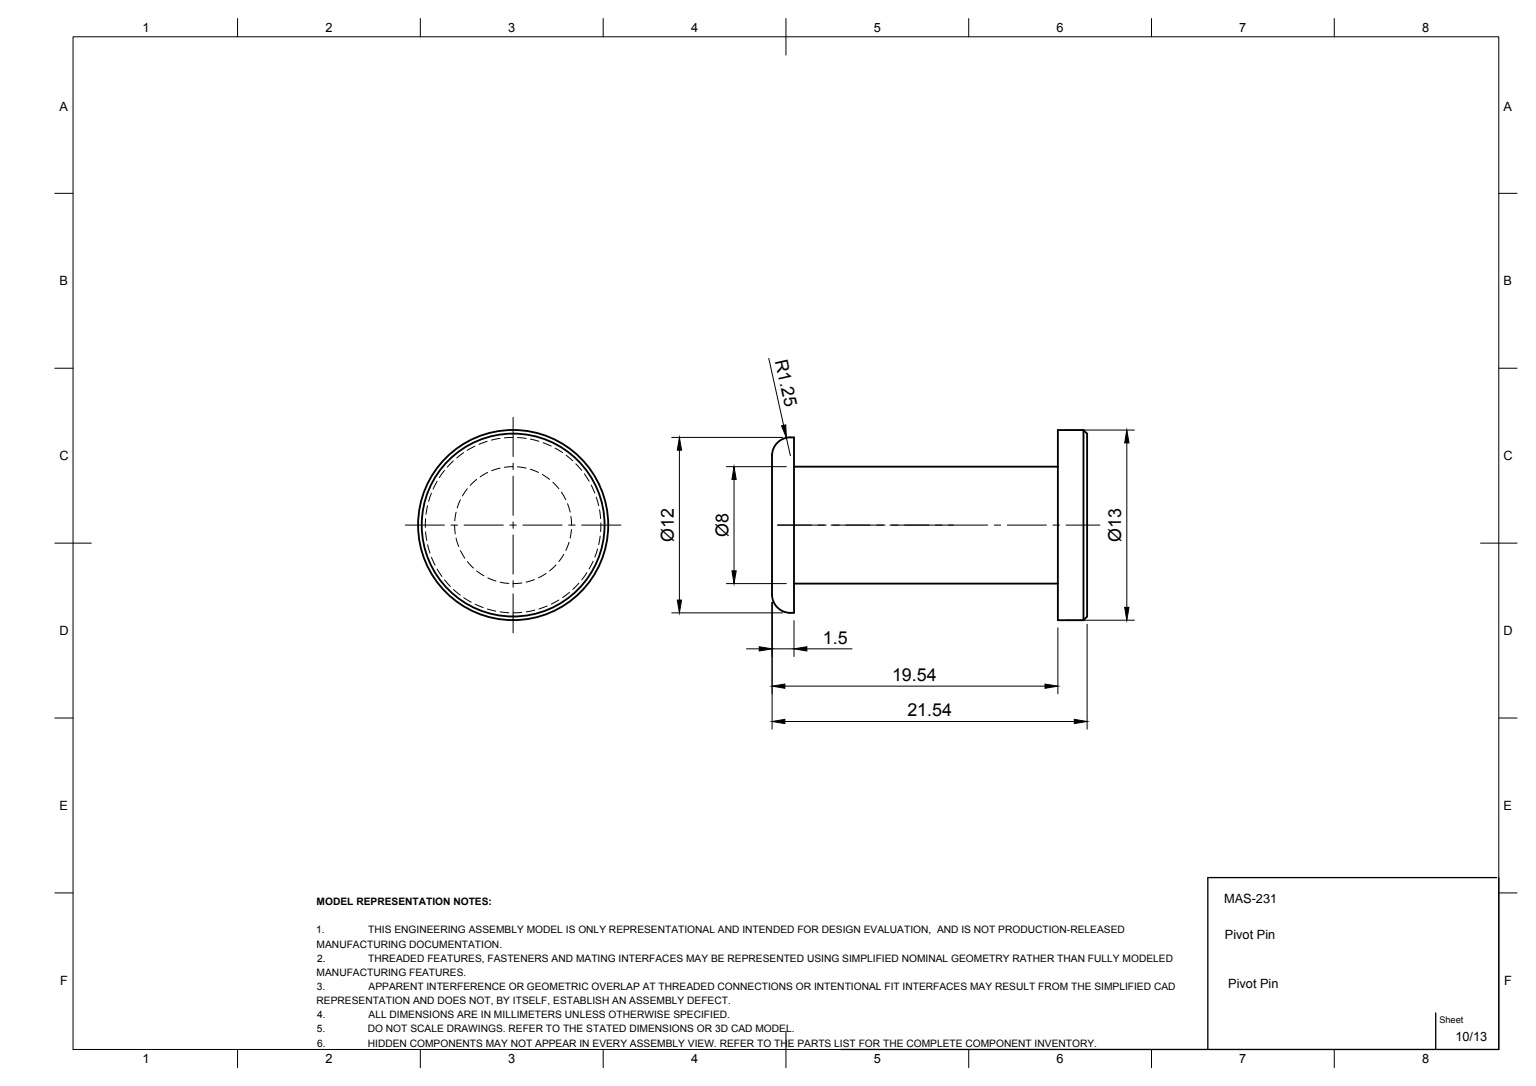
ISO-10303-21;
HEADER;
FILE_DESCRIPTION (('STEP AP214'),
    '1' );
FILE_NAME ( 'Pivot Pin.step', '2026-10-04T02:08:54', ( '' ), ( '' ), 'STEP AP214', 'Unspecified', '' );
FILE_SCHEMA (( 'AUTOMOTIVE_DESIGN' ));
ENDSEC;
DATA;
#124=DIRECTION ( 'NONE',  ( -1.000000000000000000, -6.679788269418529283E-17, 0.000000000000000000 ) ) ;
#252=CARTESIAN_POINT ( 'NONE',  ( -0.4338976377952755703, 0.1574803149606299191, 1.928577636452523993E-17 ) ) ;
#331=CIRCLE ( 'NONE', #19461, 0.1870078740157480324 ) ;
#347=EDGE_LOOP ( 'NONE', ( #1174, #678, #18238, #19385 ) ) ;
#391=FACE_OUTER_BOUND ( 'NONE', #347, .T. ) ;
#458=UNCERTAINTY_MEASURE_WITH_UNIT (LENGTH_MEASURE( 1.000000000000000082E-05 ), #21946, 'distance_accuracy_value', 'NONE') ;
#502=DIRECTION ( 'NONE',  ( 0.000000000000000000, -1.000000000000000000, 0.000000000000000000 ) ) ;
#653=ADVANCED_FACE ( 'NONE', ( #8542 ), #25959, .T. ) ;
#678=ORIENTED_EDGE ( 'NONE', *, *, #20325, .T. ) ;
#782=CARTESIAN_POINT ( 'NONE',  ( -0.3551574803149606385, -0.2559055118110236116, 0.000000000000000000 ) ) ;
#848=ADVANCED_FACE ( 'NONE', ( #29928 ), #26313, .T. ) ;
#1077=CARTESIAN_POINT ( 'NONE',  ( 0.3649999999999999911, -0.1870078740157480324, 0.000000000000000000 ) ) ;
#1174=ORIENTED_EDGE ( 'NONE', *, *, #26040, .T. ) ;
#1469=AXIS2_PLACEMENT_3D ( 'NONE', #15050, #30164, #26063 ) ;
#1552=CARTESIAN_POINT ( 'NONE',  ( -0.4338976377952755703, -2.656856766417909227E-17, 0.000000000000000000 ) ) ;
#1643=DIRECTION ( 'NONE',  ( 0.000000000000000000, -1.000000000000000000, 0.000000000000000000 ) ) ;
#1709=FACE_OUTER_BOUND ( 'NONE', #29645, .T. ) ;
#1849=DIRECTION ( 'NONE',  ( 0.000000000000000000, -1.000000000000000000, 0.000000000000000000 ) ) ;
#1886=CARTESIAN_POINT ( 'NONE',  ( -0.3551574803149606385, -2.130889186148732174E-17, 0.000000000000000000 ) ) ;
#2147=ADVANCED_BREP_SHAPE_REPRESENTATION ( 'Pivot Pin', ( #20948, #20860 ), #10178 ) ;
#2188=AXIS2_PLACEMENT_3D ( 'NONE', #20786, #27796, #9553 ) ;
#2330=DIRECTION ( 'NONE',  ( -6.679788269418529283E-17, 1.000000000000000000, 0.000000000000000000 ) ) ;
#2347=DIRECTION ( 'NONE',  ( -1.000000000000000000, 0.000000000000000000, 0.000000000000000000 ) ) ;
#2699=EDGE_CURVE ( 'NONE', #47016, #17121, #46197, .T. ) ;
#3058=ORIENTED_EDGE ( 'NONE', *, *, #38098, .F. ) ;
#3148=CARTESIAN_POINT ( 'NONE',  ( -0.3551574803149606385, -2.130889186148732174E-17, 0.000000000000000000 ) ) ;
#3307=ORIENTED_EDGE ( 'NONE', *, *, #17583, .F. ) ;
#3313=ADVANCED_FACE ( 'NONE', ( #391 ), #35406, .T. ) ;
#3390=DIRECTION ( 'NONE',  ( -1.000000000000000000, -6.679788269418529283E-17, 0.000000000000000000 ) ) ;
#3495=FILL_AREA_STYLE_COLOUR ( '', #6981 ) ;
#3752=DIRECTION ( 'NONE',  ( -6.679788269418529283E-17, 1.000000000000000000, 0.000000000000000000 ) ) ;
#3794=ADVANCED_FACE ( 'NONE', ( #5222 ), #18951, .T. ) ;
#4209=AXIS2_PLACEMENT_3D ( 'NONE', #9083, #5720, #1643 ) ;
#4634=DIRECTION ( 'NONE',  ( -1.000000000000000000, 0.000000000000000000, 0.000000000000000000 ) ) ;
#4713=VECTOR ( 'NONE', #3390, 39.37007874015748143 ) ;
#4734=DIRECTION ( 'NONE',  ( 0.000000000000000000, -1.000000000000000000, 0.000000000000000000 ) ) ;
#4837=FACE_OUTER_BOUND ( 'NONE', #10620, .T. ) ;
#4872=CARTESIAN_POINT ( 'NONE',  ( 0.3551574803149606385, 0.2362204724409449064, 2.892866454678787531E-17 ) ) ;
#5049=CARTESIAN_POINT ( 'NONE',  ( -0.3551574803149606385, -2.130889186148732174E-17, 0.000000000000000000 ) ) ;
#5182=EDGE_CURVE ( 'NONE', #17013, #26517, #16474, .T. ) ;
#5222=FACE_OUTER_BOUND ( 'NONE', #34751, .T. ) ;
#5317=DIRECTION ( 'NONE',  ( -6.679788269418529283E-17, 1.000000000000000000, 0.000000000000000000 ) ) ;
#5454=CARTESIAN_POINT ( 'NONE',  ( 0.4142125984251969206, 0.1870078740157480324, 2.591526198983078750E-17 ) ) ;
#5491=VERTEX_POINT ( 'NONE', #36851 ) ;
#5603=CARTESIAN_POINT ( 'NONE',  ( -0.3551574803149606385, 0.2559055118110236116, 3.133938659235350488E-17 ) ) ;
#5720=DIRECTION ( 'NONE',  ( -1.000000000000000000, 0.000000000000000000, 0.000000000000000000 ) ) ;
#5920=CARTESIAN_POINT ( 'NONE',  ( -0.4338976377952755703, -2.656856766417909227E-17, 0.000000000000000000 ) ) ;
#6186=ORIENTED_EDGE ( 'NONE', *, *, #12845, .F. ) ;
#6353=ORIENTED_EDGE ( 'NONE', *, *, #7044, .T. ) ;
#6396=FACE_BOUND ( 'NONE', #6977, .T. ) ;
#6432=DIRECTION ( 'NONE',  ( 0.000000000000000000, -1.000000000000000000, 0.000000000000000000 ) ) ;
#6605=( NAMED_UNIT ( * ) SI_UNIT ( $, .STERADIAN. ) SOLID_ANGLE_UNIT ( ) ) ;
#6663=VERTEX_POINT ( 'NONE', #20062 ) ;
#6696=ADVANCED_FACE ( 'NONE', ( #35411 ), #34705, .T. ) ;
#6794=ORIENTED_EDGE ( 'NONE', *, *, #27034, .F. ) ;
#6977=EDGE_LOOP ( 'NONE', ( #12832, #18302 ) ) ;
#6981=COLOUR_RGB ( '', 0.66274510, 0.83137255, 0.94901961) ;
#7044=EDGE_CURVE ( 'NONE', #6663, #21819, #18698, .T. ) ;
#7048=AXIS2_PLACEMENT_3D ( 'NONE', #29618, #25521, #44159 ) ;
#7204=LINE ( 'NONE', #36453, #18217 ) ;
#7348=APPLICATION_CONTEXT ( 'automotive_design' ) ;
#7408=ORIENTED_EDGE ( 'NONE', *, *, #36911, .T. ) ;
#7437=AXIS2_PLACEMENT_3D ( 'NONE', #1886, #16521, #31150 ) ;
#7476=DIRECTION ( 'NONE',  ( 0.000000000000000000, -1.000000000000000000, 0.000000000000000000 ) ) ;
#7557=DIRECTION ( 'NONE',  ( 0.000000000000000000, 1.000000000000000000, 0.000000000000000000 ) ) ;
#7735=AXIS2_PLACEMENT_3D ( 'NONE', #5049, #12259, #15147 ) ;
#7786=ORIENTED_EDGE ( 'NONE', *, *, #23827, .F. ) ;
#7820=VECTOR ( 'NONE', #39574, 39.37007874015748143 ) ;
#8032=AXIS2_PLACEMENT_3D ( 'NONE', #19929, #16364, #7557 ) ;
#8040=CYLINDRICAL_SURFACE ( 'NONE', #25376, 0.2559055118110236116 ) ;
#8049=PLANE ( 'NONE',  #33253 ) ;
#8122=ADVANCED_FACE ( 'NONE', ( #4837 ), #14929, .T. ) ;
#8144=VERTEX_POINT ( 'NONE', #19459 ) ;
#8204=CARTESIAN_POINT ( 'NONE',  ( -0.4338976377952755703, 5.489612613713267203E-34, 0.000000000000000000 ) ) ;
#8297=ORIENTED_EDGE ( 'NONE', *, *, #46580, .T. ) ;
#8542=FACE_OUTER_BOUND ( 'NONE', #39707, .T. ) ;
#8782=CARTESIAN_POINT ( 'NONE',  ( -0.4240551181102362177, -2.591110818884263559E-17, 0.000000000000000000 ) ) ;
#9083=CARTESIAN_POINT ( 'NONE',  ( -0.4338976377952755703, -2.656856766417909227E-17, 0.000000000000000000 ) ) ;
#9313=CARTESIAN_POINT ( 'NONE',  ( -0.4338976377952755703, -2.656856766417909227E-17, 0.000000000000000000 ) ) ;
#9553=DIRECTION ( 'NONE',  ( 6.679788269418529283E-17, -1.000000000000000000, 0.000000000000000000 ) ) ;
#9763=CARTESIAN_POINT ( 'NONE',  ( 0.3551574803149606385, -0.1574803149606299191, 0.000000000000000000 ) ) ;
#9777=PLANE ( 'NONE',  #27130 ) ;
#9906=FACE_OUTER_BOUND ( 'NONE', #18880, .T. ) ;
#10022=DIRECTION ( 'NONE',  ( 0.7071067811865450192, -0.7071067811865500152, 8.659560562354959975E-17 ) ) ;
#10178=( GEOMETRIC_REPRESENTATION_CONTEXT ( 3 ) GLOBAL_UNCERTAINTY_ASSIGNED_CONTEXT ( ( #42710 ) ) GLOBAL_UNIT_ASSIGNED_CONTEXT ( ( #26645, #38118, #23027 ) ) REPRESENTATION_CONTEXT ( 'NONE', 'WORKASPACE' ) ) ;
#10183=EDGE_CURVE ( 'NONE', #33815, #26576, #28117, .T. ) ;
#10251=FACE_OUTER_BOUND ( 'NONE', #10712, .T. ) ;
#10597=ORIENTED_EDGE ( 'NONE', *, *, #26040, .F. ) ;
#10598=AXIS2_PLACEMENT_3D ( 'NONE', #30908, #45951, #12925 ) ;
#10614=CARTESIAN_POINT ( 'NONE',  ( 0.4142125984251969206, 3.008340040661385896E-17, 0.000000000000000000 ) ) ;
#10620=EDGE_LOOP ( 'NONE', ( #3058, #29074, #26688, #21328 ) ) ;
#10712=EDGE_LOOP ( 'NONE', ( #16886, #31747 ) ) ;
#10835=DIRECTION ( 'NONE',  ( 1.000000000000000000, 0.000000000000000000, 0.000000000000000000 ) ) ;
#10990=EDGE_CURVE ( 'NONE', #5491, #44801, #14365, .T. ) ;
#11096=CARTESIAN_POINT ( 'NONE',  ( -0.4338976377952755703, -2.656856766417909227E-17, 0.000000000000000000 ) ) ;
#11101=ORIENTED_EDGE ( 'NONE', *, *, #22672, .F. ) ;
#11579=EDGE_LOOP ( 'NONE', ( #11807, #7408, #6353, #12227 ) ) ;
#11805=DIRECTION ( 'NONE',  ( -1.000000000000000000, 0.000000000000000000, 0.000000000000000000 ) ) ;
#11807=ORIENTED_EDGE ( 'NONE', *, *, #20325, .F. ) ;
#11878=EDGE_CURVE ( 'NONE', #26517, #17121, #7204, .T. ) ;
#11913=DIRECTION ( 'NONE',  ( -1.000000000000000000, -6.679788269418529283E-17, 0.000000000000000000 ) ) ;
#11945=CARTESIAN_POINT ( 'NONE',  ( 0.3551574803149606385, -0.2362204724409449064, 0.000000000000000000 ) ) ;
#11964=CARTESIAN_POINT ( 'NONE',  ( -0.3551574803149606385, -2.130889186148732174E-17, 0.000000000000000000 ) ) ;
#12227=ORIENTED_EDGE ( 'NONE', *, *, #16063, .F. ) ;
#12259=DIRECTION ( 'NONE',  ( -1.000000000000000000, 0.000000000000000000, 0.000000000000000000 ) ) ;
#12367=EDGE_CURVE ( 'NONE', #21819, #8144, #41163, .T. ) ;
#12546=DIRECTION ( 'NONE',  ( 1.000000000000000000, 6.679788269418529283E-17, 0.000000000000000000 ) ) ;
#12683=EDGE_CURVE ( 'NONE', #44801, #26576, #20119, .T. ) ;
#12832=ORIENTED_EDGE ( 'NONE', *, *, #42819, .T. ) ;
#12845=EDGE_CURVE ( 'NONE', #17121, #25548, #33566, .T. ) ;
#12900=AXIS2_PLACEMENT_3D ( 'NONE', #24429, #32096, #43331 ) ;
#12925=DIRECTION ( 'NONE',  ( 0.000000000000000000, -1.000000000000000000, 0.000000000000000000 ) ) ;
#12931=TOROIDAL_SURFACE ( 'NONE', #2188, 0.1870078740157480324, 0.04921259842519685318 ) ;
#13336=DIRECTION ( 'NONE',  ( 8.180381323125439611E-33, -1.224646799147353947E-16, 1.000000000000000000 ) ) ;
#13454=CIRCLE ( 'NONE', #35630, 0.1574803149606299191 ) ;
#13636=EDGE_CURVE ( 'NONE', #8144, #28387, #39663, .T. ) ;
#13713=AXIS2_PLACEMENT_3D ( 'NONE', #39114, #35550, #29584 ) ;
#14044=CARTESIAN_POINT ( 'NONE',  ( -0.4240551181102362177, -2.591110818884263559E-17, 0.000000000000000000 ) ) ;
#14094=CARTESIAN_POINT ( 'NONE',  ( -0.4240551181102362177, -0.2559055118110236116, 3.133938659235354185E-17 ) ) ;
#14182=ORIENTED_EDGE ( 'NONE', *, *, #12683, .F. ) ;
#14237=SHAPE_REPRESENTATION ( 'Pivot Pin', ( #20860 ), #10178 ) ;
#14290=DIRECTION ( 'NONE',  ( -1.000000000000000000, 0.000000000000000000, 0.000000000000000000 ) ) ;
#14365=CIRCLE ( 'NONE', #41097, 0.1574803149606299191 ) ;
#14462=PRODUCT_DEFINITION_CONTEXT ( 'detailed design', #7348, 'design' ) ;
#14506=ADVANCED_FACE ( 'NONE', ( #26686 ), #15900, .F. ) ;
#14512=ORIENTED_EDGE ( 'NONE', *, *, #23827, .T. ) ;
#14523=FILL_AREA_STYLE ('',( #3495 ) ) ;
#14548=DIRECTION ( 'NONE',  ( -1.000000000000000000, -6.679788269418529283E-17, 0.000000000000000000 ) ) ;
#14714=CIRCLE ( 'NONE', #24667, 0.1870078740157480324 ) ;
#14929=CONICAL_SURFACE ( 'NONE', #8032, 0.2559055118110236116, 0.7853981633974518317 ) ;
#15050=CARTESIAN_POINT ( 'NONE',  ( -0.4338976377952755703, -2.656856766417909227E-17, 0.000000000000000000 ) ) ;
#15052=APPLICATION_CONTEXT ( 'automotive_design' ) ;
#15147=DIRECTION ( 'NONE',  ( 0.000000000000000000, -1.000000000000000000, 0.000000000000000000 ) ) ;
#15223=CARTESIAN_POINT ( 'NONE',  ( -0.4338976377952755703, -0.2362204724409449064, 0.000000000000000000 ) ) ;
#15276=ADVANCED_FACE ( 'NONE', ( #1709 ), #24249, .T. ) ;
#15740=DIRECTION ( 'NONE',  ( 0.000000000000000000, 0.000000000000000000, -1.000000000000000000 ) ) ;
#15855=VERTEX_POINT ( 'NONE', #23967 ) ;
#15900=PLANE ( 'NONE',  #25196 ) ;
#15976=AXIS2_PLACEMENT_3D ( 'NONE', #40488, #36926, #21837 ) ;
#15995=ORIENTED_EDGE ( 'NONE', *, *, #10990, .F. ) ;
#16063=EDGE_CURVE ( 'NONE', #8144, #21819, #17627, .T. ) ;
#16364=DIRECTION ( 'NONE',  ( 1.000000000000000000, 0.000000000000000000, 0.000000000000000000 ) ) ;
#16457=CARTESIAN_POINT ( 'NONE',  ( 0.3649999999999999911, 0.1870078740157480324, 2.290185943287374283E-17 ) ) ;
#16474=CIRCLE ( 'NONE', #24143, 0.2559055118110236116 ) ;
#16521=DIRECTION ( 'NONE',  ( -1.000000000000000000, 0.000000000000000000, 0.000000000000000000 ) ) ;
#16674=DIRECTION ( 'NONE',  ( -1.000000000000000000, 0.000000000000000000, 0.000000000000000000 ) ) ;
#16886=ORIENTED_EDGE ( 'NONE', *, *, #27034, .T. ) ;
#16980=CARTESIAN_POINT ( 'NONE',  ( -0.4338976377952755703, -2.656856766417909227E-17, 0.000000000000000000 ) ) ;
#17013=VERTEX_POINT ( 'NONE', #5603 ) ;
#17121=VERTEX_POINT ( 'NONE', #19743 ) ;
#17488=CARTESIAN_POINT ( 'NONE',  ( -0.4240551181102362177, 0.2559055118110236116, 0.000000000000000000 ) ) ;
#17583=EDGE_CURVE ( 'NONE', #26517, #17013, #43685, .T. ) ;
#17627=CIRCLE ( 'NONE', #46690, 0.2362204724409449064 ) ;
#17771=DIRECTION ( 'NONE',  ( 0.000000000000000000, -1.000000000000000000, 0.000000000000000000 ) ) ;
#17783=CARTESIAN_POINT ( 'NONE',  ( -0.4338976377952755703, 0.2559055118110236116, 3.133938659235350488E-17 ) ) ;
#17834=CIRCLE ( 'NONE', #27026, 0.2460629921259842590 ) ;
#17897=ORIENTED_EDGE ( 'NONE', *, *, #11878, .T. ) ;
#17952=VECTOR ( 'NONE', #39988, 39.37007874015748143 ) ;
#17998=EDGE_LOOP ( 'NONE', ( #3307, #47300 ) ) ;
#18217=VECTOR ( 'NONE', #21826, 39.37007874015748143 ) ;
#18238=ORIENTED_EDGE ( 'NONE', *, *, #12367, .F. ) ;
#18302=ORIENTED_EDGE ( 'NONE', *, *, #10183, .T. ) ;
#18369=PRODUCT_DEFINITION ( 'UNKNOWN', '', #37747, #14462 ) ;
#18375=CARTESIAN_POINT ( 'NONE',  ( 0.3551574803149606385, 8.783380181941220341E-34, 0.000000000000000000 ) ) ;
#18698=CIRCLE ( 'NONE', #29581, 0.04921259842519682542 ) ;
#18880=EDGE_LOOP ( 'NONE', ( #45403, #35109, #42956, #26285 ) ) ;
#18951=CYLINDRICAL_SURFACE ( 'NONE', #27804, 0.2362204724409449064 ) ;
#19228=MECHANICAL_DESIGN_GEOMETRIC_PRESENTATION_REPRESENTATION('',(#28463),#41395);
#19385=ORIENTED_EDGE ( 'NONE', *, *, #7044, .F. ) ;
#19459=CARTESIAN_POINT ( 'NONE',  ( 0.3649999999999999911, 0.2362204724409449064, 2.892866454678787531E-17 ) ) ;
#19461=AXIS2_PLACEMENT_3D ( 'NONE', #43226, #16674, #20719 ) ;
#19658=ORIENTED_EDGE ( 'NONE', *, *, #20676, .T. ) ;
#19743=CARTESIAN_POINT ( 'NONE',  ( -0.4240551181102362177, -0.2559055118110236116, 0.000000000000000000 ) ) ;
#19825=AXIS2_PLACEMENT_3D ( 'NONE', #8782, #31323, #34677 ) ;
#19929=CARTESIAN_POINT ( 'NONE',  ( -0.4240551181102362177, -2.591110818884263559E-17, 0.000000000000000000 ) ) ;
#20062=CARTESIAN_POINT ( 'NONE',  ( 0.4142125984251969206, -0.1870078740157480324, 0.000000000000000000 ) ) ;
#20098=FACE_OUTER_BOUND ( 'NONE', #40600, .T. ) ;
#20119=LINE ( 'NONE', #34766, #44257 ) ;
#20186=SHAPE_DEFINITION_REPRESENTATION ( #30063, #14237 ) ;
#20325=EDGE_CURVE ( 'NONE', #43060, #8144, #33776, .T. ) ;
#20676=EDGE_CURVE ( 'NONE', #21819, #24360, #26728, .T. ) ;
#20719=DIRECTION ( 'NONE',  ( 0.000000000000000000, -1.000000000000000000, 0.000000000000000000 ) ) ;
#20786=CARTESIAN_POINT ( 'NONE',  ( 0.3649999999999999911, 3.414809992080327174E-17, 0.000000000000000000 ) ) ;
#20860=AXIS2_PLACEMENT_3D ( 'NONE', #25692, #32652, #10835 ) ;
#20948=MANIFOLD_SOLID_BREP ( 'Pivot Pin', #45396 ) ;
#21081=EDGE_CURVE ( 'NONE', #25548, #17121, #43710, .T. ) ;
#21328=ORIENTED_EDGE ( 'NONE', *, *, #26606, .F. ) ;
#21455=DIRECTION ( 'NONE',  ( 0.000000000000000000, -1.000000000000000000, 0.000000000000000000 ) ) ;
#21558=CARTESIAN_POINT ( 'NONE',  ( -0.3551574803149606385, -0.1574803149606299191, 0.000000000000000000 ) ) ;
#21819=VERTEX_POINT ( 'NONE', #47079 ) ;
#21826=DIRECTION ( 'NONE',  ( -1.000000000000000000, -6.679788269418529283E-17, 0.000000000000000000 ) ) ;
#21837=DIRECTION ( 'NONE',  ( 0.000000000000000000, -1.000000000000000000, 0.000000000000000000 ) ) ;
#21946=( CONVERSION_BASED_UNIT ( 'INCH', #39651 ) LENGTH_UNIT ( ) NAMED_UNIT ( #24046 ) ) ;
#22328=CARTESIAN_POINT ( 'NONE',  ( 0.3551574803149606385, 2.613864355459500179E-17, 0.000000000000000000 ) ) ;
#22366=AXIS2_PLACEMENT_3D ( 'NONE', #22328, #11805, #7476 ) ;
#22611=PRODUCT_CONTEXT ( 'NONE', #15052, 'mechanical' ) ;
#22668=DIRECTION ( 'NONE',  ( 0.000000000000000000, -1.000000000000000000, 0.000000000000000000 ) ) ;
#22672=EDGE_CURVE ( 'NONE', #44801, #5491, #46863, .T. ) ;
#23027=( NAMED_UNIT ( * ) SI_UNIT ( $, .STERADIAN. ) SOLID_ANGLE_UNIT ( ) ) ;
#23185=ORIENTED_EDGE ( 'NONE', *, *, #36437, .T. ) ;
#23827=EDGE_CURVE ( 'NONE', #15855, #47016, #17834, .T. ) ;
#23936=DIRECTION ( 'NONE',  ( 0.000000000000000000, -1.000000000000000000, 0.000000000000000000 ) ) ;
#23967=CARTESIAN_POINT ( 'NONE',  ( -0.4338976377952755703, 0.2460629921259842590, 0.000000000000000000 ) ) ;
#24046=DIMENSIONAL_EXPONENTS ( 1.000000000000000000, 0.000000000000000000, 0.000000000000000000, 0.000000000000000000, 0.000000000000000000, 0.000000000000000000, 0.000000000000000000 ) ;
#24143=AXIS2_PLACEMENT_3D ( 'NONE', #11964, #37574, #4734 ) ;
#24249=PLANE ( 'NONE',  #42064 ) ;
#24326=PRODUCT ( 'Pivot Pin', 'Pivot Pin', '', ( #22611 ) ) ;
#24360=VERTEX_POINT ( 'NONE', #11945 ) ;
#24429=CARTESIAN_POINT ( 'NONE',  ( -0.4240551181102362177, -2.591110818884263559E-17, 0.000000000000000000 ) ) ;
#24516=CYLINDRICAL_SURFACE ( 'NONE', #13713, 0.1574803149606299191 ) ;
#24636=CARTESIAN_POINT ( 'NONE',  ( -0.3551574803149606385, 0.1574803149606299191, 1.928577636452523993E-17 ) ) ;
#24667=AXIS2_PLACEMENT_3D ( 'NONE', #10614, #43885, #29342 ) ;
#24823=( LENGTH_UNIT ( ) NAMED_UNIT ( * ) SI_UNIT ( $, .METRE. ) ) ;
#24907=CIRCLE ( 'NONE', #4209, 0.2460629921259842590 ) ;
#24980=LINE ( 'NONE', #17783, #7820 ) ;
#25090=FACE_OUTER_BOUND ( 'NONE', #17998, .T. ) ;
#25196=AXIS2_PLACEMENT_3D ( 'NONE', #8204, #12546, #5317 ) ;
#25376=AXIS2_PLACEMENT_3D ( 'NONE', #1552, #41548, #22668 ) ;
#25377=AXIS2_PLACEMENT_3D ( 'NONE', #14044, #14290, #21455 ) ;
#25383=DIRECTION ( 'NONE',  ( -1.000000000000000000, 0.000000000000000000, 0.000000000000000000 ) ) ;
#25521=DIRECTION ( 'NONE',  ( -1.000000000000000000, 0.000000000000000000, 0.000000000000000000 ) ) ;
#25548=VERTEX_POINT ( 'NONE', #39456 ) ;
#25582=ORIENTED_EDGE ( 'NONE', *, *, #36437, .F. ) ;
#25626=ADVANCED_FACE ( 'NONE', ( #6396, #25090 ), #9777, .F. ) ;
#25668=ADVANCED_FACE ( 'NONE', ( #46646, #10251 ), #8049, .T. ) ;
#25692=CARTESIAN_POINT ( 'NONE',  ( 0.000000000000000000, 0.000000000000000000, 0.000000000000000000 ) ) ;
#25719=DIRECTION ( 'NONE',  ( -1.000000000000000000, 0.000000000000000000, 0.000000000000000000 ) ) ;
#25890=EDGE_LOOP ( 'NONE', ( #25582, #43075, #17897, #36868 ) ) ;
#25914=ORIENTED_EDGE ( 'NONE', *, *, #42819, .F. ) ;
#25959=CONICAL_SURFACE ( 'NONE', #19825, 0.2559055118110236116, 0.7853981633974518317 ) ;
#26040=EDGE_CURVE ( 'NONE', #6663, #43060, #331, .T. ) ;
#26063=DIRECTION ( 'NONE',  ( 0.000000000000000000, -1.000000000000000000, 0.000000000000000000 ) ) ;
#26117=AXIS2_PLACEMENT_3D ( 'NONE', #16457, #13336, #30860 ) ;
#26224=CIRCLE ( 'NONE', #7048, 0.2362204724409449064 ) ;
#26285=ORIENTED_EDGE ( 'NONE', *, *, #10183, .F. ) ;
#26313=CYLINDRICAL_SURFACE ( 'NONE', #1469, 0.2559055118110236116 ) ;
#26517=VERTEX_POINT ( 'NONE', #782 ) ;
#26576=VERTEX_POINT ( 'NONE', #21558 ) ;
#26606=EDGE_CURVE ( 'NONE', #15855, #25548, #27435, .T. ) ;
#26645=( CONVERSION_BASED_UNIT ( 'INCH', #38343 ) LENGTH_UNIT ( ) NAMED_UNIT ( #35386 ) ) ;
#26686=FACE_OUTER_BOUND ( 'NONE', #27287, .T. ) ;
#26688=ORIENTED_EDGE ( 'NONE', *, *, #12845, .T. ) ;
#26728=LINE ( 'NONE', #15223, #38349 ) ;
#27016=DIRECTION ( 'NONE',  ( 6.679788269418529283E-17, -1.000000000000000000, 0.000000000000000000 ) ) ;
#27026=AXIS2_PLACEMENT_3D ( 'NONE', #11096, #25719, #502 ) ;
#27034=EDGE_CURVE ( 'NONE', #24360, #28387, #36615, .T. ) ;
#27130=AXIS2_PLACEMENT_3D ( 'NONE', #42569, #28474, #2330 ) ;
#27287=EDGE_LOOP ( 'NONE', ( #14512, #34743 ) ) ;
#27435=LINE ( 'NONE', #17488, #17952 ) ;
#27477=ORIENTED_EDGE ( 'NONE', *, *, #22672, .T. ) ;
#27796=DIRECTION ( 'NONE',  ( -1.000000000000000000, -6.679788269418529283E-17, 0.000000000000000000 ) ) ;
#27804=AXIS2_PLACEMENT_3D ( 'NONE', #9313, #34478, #23936 ) ;
#28117=CIRCLE ( 'NONE', #7437, 0.1574803149606299191 ) ;
#28387=VERTEX_POINT ( 'NONE', #4872 ) ;
#28463=STYLED_ITEM ( 'NONE', ( #43260 ), #20948 ) ;
#28474=DIRECTION ( 'NONE',  ( -1.000000000000000000, -6.679788269418529283E-17, 0.000000000000000000 ) ) ;
#28767=ADVANCED_FACE ( 'NONE', ( #9906 ), #24516, .T. ) ;
#28830=ORIENTED_EDGE ( 'NONE', *, *, #2699, .F. ) ;
#29074=ORIENTED_EDGE ( 'NONE', *, *, #2699, .T. ) ;
#29220=VECTOR ( 'NONE', #10022, 39.37007874015748143 ) ;
#29230=EDGE_LOOP ( 'NONE', ( #11101, #15995 ) ) ;
#29266=ORIENTED_EDGE ( 'NONE', *, *, #13636, .T. ) ;
#29342=DIRECTION ( 'NONE',  ( 0.000000000000000000, -1.000000000000000000, 0.000000000000000000 ) ) ;
#29581=AXIS2_PLACEMENT_3D ( 'NONE', #1077, #15740, #34187 ) ;
#29584=DIRECTION ( 'NONE',  ( 0.000000000000000000, -1.000000000000000000, 0.000000000000000000 ) ) ;
#29618=CARTESIAN_POINT ( 'NONE',  ( 0.3551574803149606385, 2.613864355459500179E-17, 0.000000000000000000 ) ) ;
#29645=EDGE_LOOP ( 'NONE', ( #10597, #46195 ) ) ;
#29928=FACE_OUTER_BOUND ( 'NONE', #25890, .T. ) ;
#30063=PRODUCT_DEFINITION_SHAPE ( 'NONE', 'NONE',  #18369 ) ;
#30164=DIRECTION ( 'NONE',  ( -1.000000000000000000, 0.000000000000000000, 0.000000000000000000 ) ) ;
#30553=EDGE_LOOP ( 'NONE', ( #43538, #23185, #6186, #39140 ) ) ;
#30559=VECTOR ( 'NONE', #124, 39.37007874015748143 ) ;
#30749=DIRECTION ( 'NONE',  ( -6.679788269418529283E-17, 1.000000000000000000, 0.000000000000000000 ) ) ;
#30840=AXIS2_PLACEMENT_3D ( 'NONE', #30850, #11913, #27016 ) ;
#30850=CARTESIAN_POINT ( 'NONE',  ( 0.3649999999999999911, 3.414809992080327174E-17, 0.000000000000000000 ) ) ;
#30860=DIRECTION ( 'NONE',  ( 0.000000000000000000, -1.000000000000000000, -1.224646799147353947E-16 ) ) ;
#30908=CARTESIAN_POINT ( 'NONE',  ( 0.3551574803149606385, 2.613864355459500179E-17, 0.000000000000000000 ) ) ;
#31150=DIRECTION ( 'NONE',  ( 0.000000000000000000, -1.000000000000000000, 0.000000000000000000 ) ) ;
#31323=DIRECTION ( 'NONE',  ( 1.000000000000000000, 0.000000000000000000, 0.000000000000000000 ) ) ;
#31389=CYLINDRICAL_SURFACE ( 'NONE', #35648, 0.2362204724409449064 ) ;
#31747=ORIENTED_EDGE ( 'NONE', *, *, #47184, .T. ) ;
#31817=DIRECTION ( 'NONE',  ( -1.000000000000000000, 0.000000000000000000, 0.000000000000000000 ) ) ;
#32096=DIRECTION ( 'NONE',  ( -1.000000000000000000, 0.000000000000000000, 0.000000000000000000 ) ) ;
#32276=SURFACE_STYLE_FILL_AREA ( #14523 ) ;
#32652=DIRECTION ( 'NONE',  ( 0.000000000000000000, 0.000000000000000000, 1.000000000000000000 ) ) ;
#33002=CARTESIAN_POINT ( 'NONE',  ( -0.4338976377952755703, 0.2362204724409449064, 2.892866454678787531E-17 ) ) ;
#33221=DIRECTION ( 'NONE',  ( -1.000000000000000000, -6.679788269418529283E-17, 0.000000000000000000 ) ) ;
#33253=AXIS2_PLACEMENT_3D ( 'NONE', #18375, #14548, #3752 ) ;
#33566=CIRCLE ( 'NONE', #12900, 0.2559055118110236116 ) ;
#33776=CIRCLE ( 'NONE', #26117, 0.04921259842519686012 ) ;
#33815=VERTEX_POINT ( 'NONE', #24636 ) ;
#33838=ORIENTED_EDGE ( 'NONE', *, *, #47184, .F. ) ;
#34076=( LENGTH_UNIT ( ) NAMED_UNIT ( * ) SI_UNIT ( $, .METRE. ) ) ;
#34187=DIRECTION ( 'NONE',  ( -1.000000000000000000, 0.000000000000000000, 0.000000000000000000 ) ) ;
#34478=DIRECTION ( 'NONE',  ( -1.000000000000000000, 0.000000000000000000, 0.000000000000000000 ) ) ;
#34648=FACE_OUTER_BOUND ( 'NONE', #30553, .T. ) ;
#34677=DIRECTION ( 'NONE',  ( 0.000000000000000000, 1.000000000000000000, 0.000000000000000000 ) ) ;
#34705=CYLINDRICAL_SURFACE ( 'NONE', #35558, 0.1574803149606299191 ) ;
#34743=ORIENTED_EDGE ( 'NONE', *, *, #38098, .T. ) ;
#34751=EDGE_LOOP ( 'NONE', ( #37548, #47421, #19658, #33838 ) ) ;
#34766=CARTESIAN_POINT ( 'NONE',  ( -0.4338976377952755703, -0.1574803149606299191, 0.000000000000000000 ) ) ;
#34780=SHAPE_REPRESENTATION_RELATIONSHIP ( 'NONE' , 'NONE' ,  #14237, #2147 ) ;
#34811=CARTESIAN_POINT ( 'NONE',  ( 0.4142125984251969206, -1.512724881123248161E-16, 0.000000000000000000 ) ) ;
#35109=ORIENTED_EDGE ( 'NONE', *, *, #10990, .T. ) ;
#35386=DIMENSIONAL_EXPONENTS ( 1.000000000000000000, 0.000000000000000000, 0.000000000000000000, 0.000000000000000000, 0.000000000000000000, 0.000000000000000000, 0.000000000000000000 ) ;
#35406=TOROIDAL_SURFACE ( 'NONE', #30840, 0.1870078740157480324, 0.04921259842519685318 ) ;
#35411=FACE_OUTER_BOUND ( 'NONE', #44047, .T. ) ;
#35441=DIRECTION ( 'NONE',  ( 0.000000000000000000, -1.000000000000000000, 0.000000000000000000 ) ) ;
#35550=DIRECTION ( 'NONE',  ( -1.000000000000000000, 0.000000000000000000, 0.000000000000000000 ) ) ;
#35558=AXIS2_PLACEMENT_3D ( 'NONE', #5920, #31817, #1849 ) ;
#35630=AXIS2_PLACEMENT_3D ( 'NONE', #3148, #35987, #17771 ) ;
#35648=AXIS2_PLACEMENT_3D ( 'NONE', #16980, #2347, #35441 ) ;
#35987=DIRECTION ( 'NONE',  ( -1.000000000000000000, 0.000000000000000000, 0.000000000000000000 ) ) ;
#36342=SURFACE_STYLE_USAGE ( .BOTH. , #43973 ) ;
#36437=EDGE_CURVE ( 'NONE', #17013, #25548, #24980, .T. ) ;
#36453=CARTESIAN_POINT ( 'NONE',  ( -0.4338976377952755703, -0.2559055118110236116, 0.000000000000000000 ) ) ;
#36615=CIRCLE ( 'NONE', #10598, 0.2362204724409449064 ) ;
#36660=ORIENTED_EDGE ( 'NONE', *, *, #26606, .T. ) ;
#36851=CARTESIAN_POINT ( 'NONE',  ( 0.3551574803149606385, 0.1574803149606299191, 1.928577636452523993E-17 ) ) ;
#36868=ORIENTED_EDGE ( 'NONE', *, *, #21081, .F. ) ;
#36911=EDGE_CURVE ( 'NONE', #43060, #6663, #14714, .T. ) ;
#36926=DIRECTION ( 'NONE',  ( -1.000000000000000000, 0.000000000000000000, 0.000000000000000000 ) ) ;
#37073=ORIENTED_EDGE ( 'NONE', *, *, #21081, .T. ) ;
#37482=CARTESIAN_POINT ( 'NONE',  ( 0.3551574803149606385, 2.613864355459500179E-17, 0.000000000000000000 ) ) ;
#37548=ORIENTED_EDGE ( 'NONE', *, *, #13636, .F. ) ;
#37574=DIRECTION ( 'NONE',  ( -1.000000000000000000, 0.000000000000000000, 0.000000000000000000 ) ) ;
#37747=PRODUCT_DEFINITION_FORMATION_WITH_SPECIFIED_SOURCE ( 'ANY', '', #24326, .NOT_KNOWN. ) ;
#38098=EDGE_CURVE ( 'NONE', #47016, #15855, #24907, .T. ) ;
#38118=( NAMED_UNIT ( * ) PLANE_ANGLE_UNIT ( ) SI_UNIT ( $, .RADIAN. ) ) ;
#38143=ADVANCED_FACE ( 'NONE', ( #20098 ), #31389, .T. ) ;
#38343=LENGTH_MEASURE_WITH_UNIT ( LENGTH_MEASURE( 0.02539999999999999897 ), #34076 ) ;
#38349=VECTOR ( 'NONE', #33221, 39.37007874015748143 ) ;
#39114=CARTESIAN_POINT ( 'NONE',  ( -0.4338976377952755703, -2.656856766417909227E-17, 0.000000000000000000 ) ) ;
#39140=ORIENTED_EDGE ( 'NONE', *, *, #11878, .F. ) ;
#39456=CARTESIAN_POINT ( 'NONE',  ( -0.4240551181102362177, 0.2559055118110236116, 3.133938659235354185E-17 ) ) ;
#39494=CARTESIAN_POINT ( 'NONE',  ( 0.3649999999999999911, 2.679610302993149545E-17, 0.000000000000000000 ) ) ;
#39574=DIRECTION ( 'NONE',  ( -1.000000000000000000, -6.679788269418529283E-17, 0.000000000000000000 ) ) ;
#39651=LENGTH_MEASURE_WITH_UNIT ( LENGTH_MEASURE( 0.02539999999999999897 ), #24823 ) ;
#39663=LINE ( 'NONE', #33002, #30559 ) ;
#39707=EDGE_LOOP ( 'NONE', ( #28830, #7786, #36660, #37073 ) ) ;
#39923=ADVANCED_FACE ( 'NONE', ( #41201 ), #12931, .T. ) ;
#39988=DIRECTION ( 'NONE',  ( 0.7071067811865450192, 0.7071067811865500152, 0.000000000000000000 ) ) ;
#40488=CARTESIAN_POINT ( 'NONE',  ( 0.3649999999999999911, 2.679610302993149545E-17, 0.000000000000000000 ) ) ;
#40600=EDGE_LOOP ( 'NONE', ( #41294, #29266, #6794, #40631 ) ) ;
#40631=ORIENTED_EDGE ( 'NONE', *, *, #20676, .F. ) ;
#41097=AXIS2_PLACEMENT_3D ( 'NONE', #37482, #4634, #44886 ) ;
#41163=CIRCLE ( 'NONE', #15976, 0.2362204724409449064 ) ;
#41201=FACE_OUTER_BOUND ( 'NONE', #11579, .T. ) ;
#41294=ORIENTED_EDGE ( 'NONE', *, *, #12367, .T. ) ;
#41395=( GEOMETRIC_REPRESENTATION_CONTEXT ( 3 ) GLOBAL_UNCERTAINTY_ASSIGNED_CONTEXT ( ( #458 ) ) GLOBAL_UNIT_ASSIGNED_CONTEXT ( ( #21946, #43010, #6605 ) ) REPRESENTATION_CONTEXT ( 'NONE', 'WORKASPACE' ) ) ;
#41548=DIRECTION ( 'NONE',  ( -1.000000000000000000, 0.000000000000000000, 0.000000000000000000 ) ) ;
#41900=DIRECTION ( 'NONE',  ( -1.000000000000000000, -6.679788269418529283E-17, 0.000000000000000000 ) ) ;
#42064=AXIS2_PLACEMENT_3D ( 'NONE', #34811, #42652, #30749 ) ;
#42569=CARTESIAN_POINT ( 'NONE',  ( -0.3551574803149606385, 9.222549191038288286E-34, 0.000000000000000000 ) ) ;
#42652=DIRECTION ( 'NONE',  ( 1.000000000000000000, 6.679788269418529283E-17, 0.000000000000000000 ) ) ;
#42710=UNCERTAINTY_MEASURE_WITH_UNIT (LENGTH_MEASURE( 1.000000000000000082E-05 ), #26645, 'distance_accuracy_value', 'NONE') ;
#42819=EDGE_CURVE ( 'NONE', #26576, #33815, #13454, .T. ) ;
#42956=ORIENTED_EDGE ( 'NONE', *, *, #12683, .T. ) ;
#43010=( NAMED_UNIT ( * ) PLANE_ANGLE_UNIT ( ) SI_UNIT ( $, .RADIAN. ) ) ;
#43060=VERTEX_POINT ( 'NONE', #5454 ) ;
#43075=ORIENTED_EDGE ( 'NONE', *, *, #5182, .T. ) ;
#43226=CARTESIAN_POINT ( 'NONE',  ( 0.4142125984251969206, 3.008340040661385896E-17, 0.000000000000000000 ) ) ;
#43260=PRESENTATION_STYLE_ASSIGNMENT (( #36342 ) ) ;
#43331=DIRECTION ( 'NONE',  ( 0.000000000000000000, -1.000000000000000000, 0.000000000000000000 ) ) ;
#43538=ORIENTED_EDGE ( 'NONE', *, *, #17583, .T. ) ;
#43685=CIRCLE ( 'NONE', #7735, 0.2559055118110236116 ) ;
#43710=CIRCLE ( 'NONE', #25377, 0.2559055118110236116 ) ;
#43885=DIRECTION ( 'NONE',  ( -1.000000000000000000, 0.000000000000000000, 0.000000000000000000 ) ) ;
#43973=SURFACE_SIDE_STYLE ('',( #32276 ) ) ;
#44047=EDGE_LOOP ( 'NONE', ( #27477, #8297, #25914, #14182 ) ) ;
#44159=DIRECTION ( 'NONE',  ( 0.000000000000000000, -1.000000000000000000, 0.000000000000000000 ) ) ;
#44257=VECTOR ( 'NONE', #41900, 39.37007874015748143 ) ;
#44457=CARTESIAN_POINT ( 'NONE',  ( -0.4338976377952755703, -0.2460629921259842590, 3.073670608096212368E-17 ) ) ;
#44801=VERTEX_POINT ( 'NONE', #9763 ) ;
#44886=DIRECTION ( 'NONE',  ( 0.000000000000000000, -1.000000000000000000, 0.000000000000000000 ) ) ;
#45396=CLOSED_SHELL ( 'NONE', ( #653, #848, #25626, #28767, #25668, #3794, #39923, #15276, #14506, #3313, #38143, #6696, #45526, #8122 ) ) ;
#45403=ORIENTED_EDGE ( 'NONE', *, *, #46580, .F. ) ;
#45526=ADVANCED_FACE ( 'NONE', ( #34648 ), #8040, .T. ) ;
#45951=DIRECTION ( 'NONE',  ( -1.000000000000000000, 0.000000000000000000, 0.000000000000000000 ) ) ;
#46195=ORIENTED_EDGE ( 'NONE', *, *, #36911, .F. ) ;
#46197=LINE ( 'NONE', #14094, #29220 ) ;
#46580=EDGE_CURVE ( 'NONE', #5491, #33815, #47239, .T. ) ;
#46646=FACE_BOUND ( 'NONE', #29230, .T. ) ;
#46690=AXIS2_PLACEMENT_3D ( 'NONE', #39494, #25383, #6432 ) ;
#46863=CIRCLE ( 'NONE', #22366, 0.1574803149606299191 ) ;
#47016=VERTEX_POINT ( 'NONE', #44457 ) ;
#47079=CARTESIAN_POINT ( 'NONE',  ( 0.3649999999999999911, -0.2362204724409449064, 0.000000000000000000 ) ) ;
#47184=EDGE_CURVE ( 'NONE', #28387, #24360, #26224, .T. ) ;
#47239=LINE ( 'NONE', #252, #4713 ) ;
#47300=ORIENTED_EDGE ( 'NONE', *, *, #5182, .F. ) ;
#47421=ORIENTED_EDGE ( 'NONE', *, *, #16063, .T. ) ;
ENDSEC;
END-ISO-10303-21;
